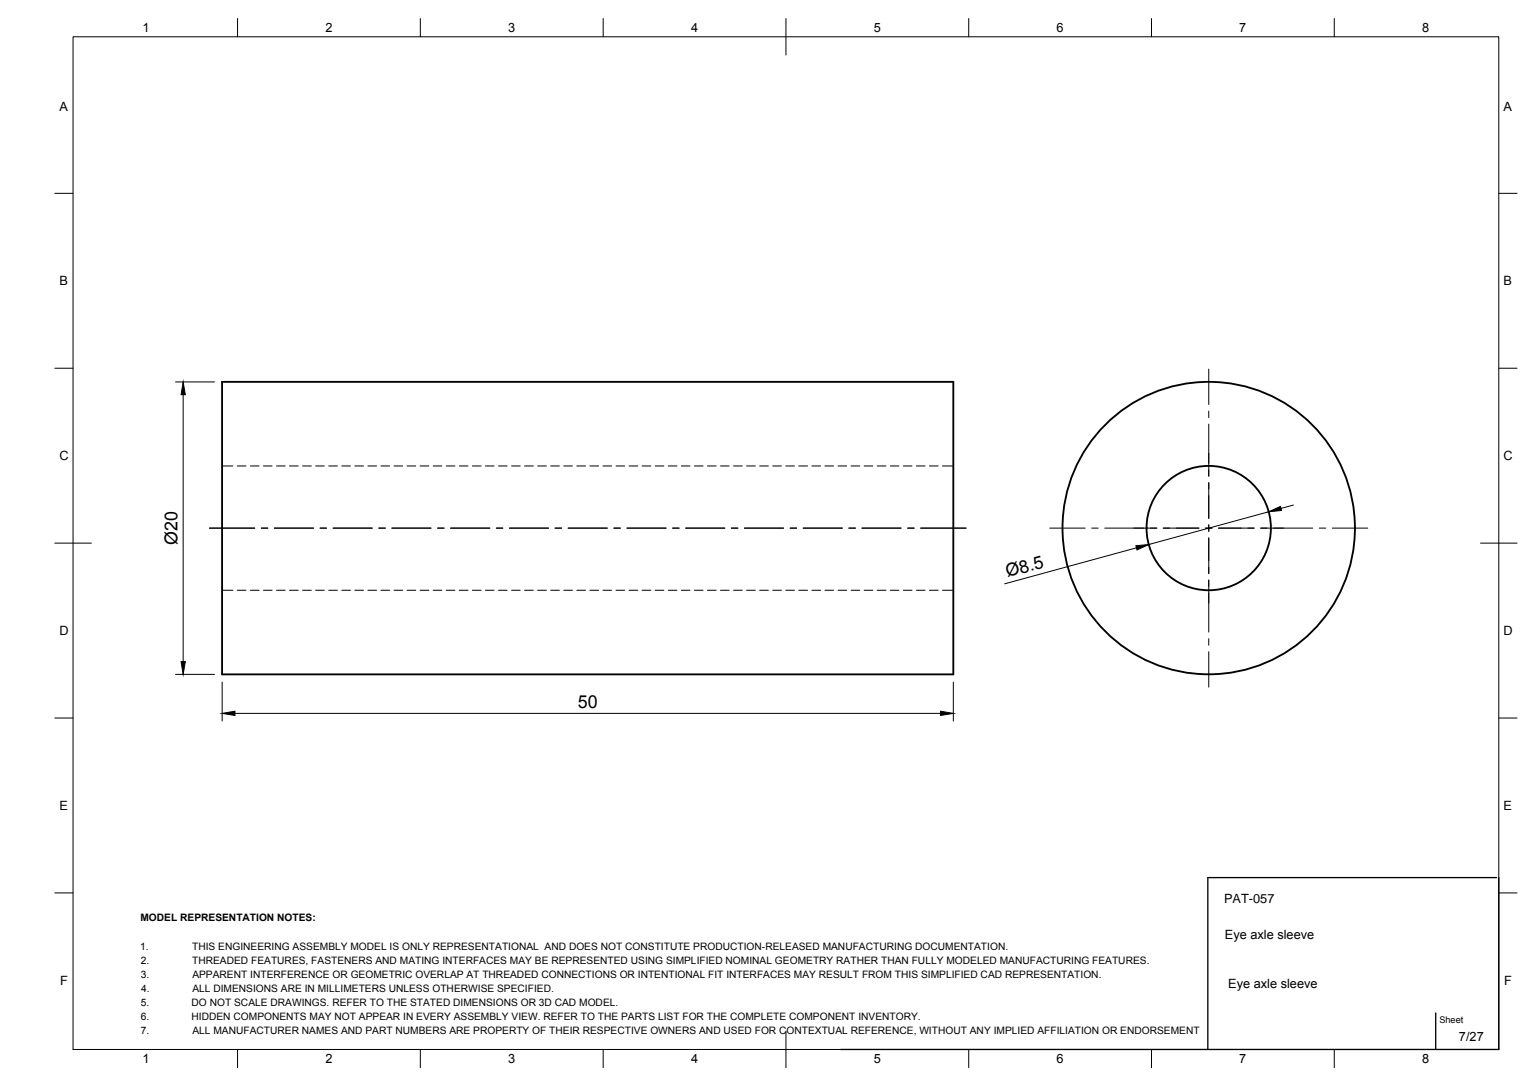
ISO-10303-21;
HEADER;
/* Generated by software containing ST-Developer
 * from STEP Tools, Inc. (www.steptools.com) 
 */

FILE_DESCRIPTION(
/* description */ ('Bearing-mounted hook block'),
/* implementation_level */ '2;1');

FILE_NAME(
/* name */ 'Eye axle sleeve.step',
/* time_stamp */ '2026-10-28T22:30:11-07:00',
/* author */ (''),
/* organization */ (''),
/* preprocessor_version */ 'ST-DEVELOPER v20.2',
/* originating_system */ 'Autodesk Translation Framework v15.17.0.0',
/* authorisation */ '');

FILE_SCHEMA (('AUTOMOTIVE_DESIGN { 1 0 10303 214 3 1 1 }'));
ENDSEC;

DATA;
#10=MECHANICAL_DESIGN_GEOMETRIC_PRESENTATION_REPRESENTATION('',(#325),#7609);
#277=SHAPE_REPRESENTATION_RELATIONSHIP('SRR','None',#7724,#301);
#301=ADVANCED_BREP_SHAPE_REPRESENTATION('',(#357),#7584);
#325=STYLED_ITEM('',(#7931),#357);
#357=MANIFOLD_SOLID_BREP('Body1',#3921);
#440=LINE('',#6266,#670);
#441=LINE('',#6272,#671);
#670=VECTOR('',#4975,0.425);
#671=VECTOR('',#4982,1.);
#860=CYLINDRICAL_SURFACE('',#4298,0.425);
#861=CYLINDRICAL_SURFACE('',#4301,1.);
#941=FACE_BOUND('',#1294,.T.);
#942=FACE_BOUND('',#1296,.T.);
#1035=FACE_OUTER_BOUND('',#1291,.T.);
#1036=FACE_OUTER_BOUND('',#1292,.T.);
#1037=FACE_OUTER_BOUND('',#1293,.T.);
#1038=FACE_OUTER_BOUND('',#1295,.T.);
#1291=EDGE_LOOP('',(#2782,#2783,#2784,#2785));
#1292=EDGE_LOOP('',(#2786,#2787,#2788,#2789));
#1293=EDGE_LOOP('',(#2790));
#1294=EDGE_LOOP('',(#2791));
#1295=EDGE_LOOP('',(#2792));
#1296=EDGE_LOOP('',(#2793));
#1593=CIRCLE('',#4299,0.425);
#1594=CIRCLE('',#4300,0.425);
#1595=CIRCLE('',#4302,1.);
#1596=CIRCLE('',#4303,1.);
#1842=VERTEX_POINT('',#6263);
#1843=VERTEX_POINT('',#6265);
#1844=VERTEX_POINT('',#6269);
#1845=VERTEX_POINT('',#6271);
#2201=EDGE_CURVE('',#1842,#1842,#1593,.T.);
#2202=EDGE_CURVE('',#1842,#1843,#440,.T.);
#2203=EDGE_CURVE('',#1843,#1843,#1594,.T.);
#2204=EDGE_CURVE('',#1844,#1844,#1595,.T.);
#2205=EDGE_CURVE('',#1844,#1845,#441,.T.);
#2206=EDGE_CURVE('',#1845,#1845,#1596,.T.);
#2782=ORIENTED_EDGE('',*,*,#2201,.F.);
#2783=ORIENTED_EDGE('',*,*,#2202,.T.);
#2784=ORIENTED_EDGE('',*,*,#2203,.T.);
#2785=ORIENTED_EDGE('',*,*,#2202,.F.);
#2786=ORIENTED_EDGE('',*,*,#2204,.F.);
#2787=ORIENTED_EDGE('',*,*,#2205,.T.);
#2788=ORIENTED_EDGE('',*,*,#2206,.T.);
#2789=ORIENTED_EDGE('',*,*,#2205,.F.);
#2790=ORIENTED_EDGE('',*,*,#2204,.T.);
#2791=ORIENTED_EDGE('',*,*,#2201,.T.);
#2792=ORIENTED_EDGE('',*,*,#2206,.F.);
#2793=ORIENTED_EDGE('',*,*,#2203,.F.);
#3578=PLANE('',#4304);
#3579=PLANE('',#4305);
#3717=ADVANCED_FACE('',(#1035),#860,.F.);
#3718=ADVANCED_FACE('',(#1036),#861,.T.);
#3719=ADVANCED_FACE('',(#1037,#941),#3578,.T.);
#3720=ADVANCED_FACE('',(#1038,#942),#3579,.F.);
#3921=CLOSED_SHELL('',(#3717,#3718,#3719,#3720));
#4297=AXIS2_PLACEMENT_3D('',#6261,#4969,#4970);
#4298=AXIS2_PLACEMENT_3D('',#6262,#4971,#4972);
#4299=AXIS2_PLACEMENT_3D('',#6264,#4973,#4974);
#4300=AXIS2_PLACEMENT_3D('',#6267,#4976,#4977);
#4301=AXIS2_PLACEMENT_3D('',#6268,#4978,#4979);
#4302=AXIS2_PLACEMENT_3D('',#6270,#4980,#4981);
#4303=AXIS2_PLACEMENT_3D('',#6273,#4983,#4984);
#4304=AXIS2_PLACEMENT_3D('',#6274,#4985,#4986);
#4305=AXIS2_PLACEMENT_3D('',#6275,#4987,#4988);
#4969=DIRECTION('axis',(0.,0.,1.));
#4970=DIRECTION('refdir',(1.,0.,0.));
#4971=DIRECTION('center_axis',(0.,1.,0.));
#4972=DIRECTION('ref_axis',(1.,0.,0.));
#4973=DIRECTION('center_axis',(0.,-1.,0.));
#4974=DIRECTION('ref_axis',(1.,0.,0.));
#4975=DIRECTION('',(0.,-1.,0.));
#4976=DIRECTION('center_axis',(0.,-1.,0.));
#4977=DIRECTION('ref_axis',(1.,0.,0.));
#4978=DIRECTION('center_axis',(0.,1.,0.));
#4979=DIRECTION('ref_axis',(1.,0.,0.));
#4980=DIRECTION('center_axis',(0.,1.,0.));
#4981=DIRECTION('ref_axis',(1.,0.,0.));
#4982=DIRECTION('',(0.,-1.,0.));
#4983=DIRECTION('center_axis',(0.,1.,0.));
#4984=DIRECTION('ref_axis',(1.,0.,0.));
#4985=DIRECTION('center_axis',(0.,1.,0.));
#4986=DIRECTION('ref_axis',(1.,0.,0.));
#4987=DIRECTION('center_axis',(0.,1.,0.));
#4988=DIRECTION('ref_axis',(1.,0.,0.));
#6261=CARTESIAN_POINT('',(0.,0.,0.));
#6262=CARTESIAN_POINT('Origin',(0.,-2.5,20.5));
#6263=CARTESIAN_POINT('',(-0.425,2.5,20.5));
#6264=CARTESIAN_POINT('Origin',(0.,2.5,20.5));
#6265=CARTESIAN_POINT('',(-0.425,-2.5,20.5));
#6266=CARTESIAN_POINT('',(-0.425,-2.5,20.5));
#6267=CARTESIAN_POINT('Origin',(0.,-2.5,20.5));
#6268=CARTESIAN_POINT('Origin',(0.,-2.5,20.5));
#6269=CARTESIAN_POINT('',(-1.,2.5,20.5));
#6270=CARTESIAN_POINT('Origin',(0.,2.5,20.5));
#6271=CARTESIAN_POINT('',(-1.,-2.5,20.5));
#6272=CARTESIAN_POINT('',(-1.,-2.5,20.5));
#6273=CARTESIAN_POINT('Origin',(0.,-2.5,20.5));
#6274=CARTESIAN_POINT('Origin',(0.,2.5,20.5));
#6275=CARTESIAN_POINT('Origin',(0.,-2.5,20.5));
#7554=UNCERTAINTY_MEASURE_WITH_UNIT(LENGTH_MEASURE(0.001),#7610,
'DISTANCE_ACCURACY_VALUE',
'Maximum model space distance between geometric entities at asserted c
onnectivities');
#7579=UNCERTAINTY_MEASURE_WITH_UNIT(LENGTH_MEASURE(0.001),#7610,
'DISTANCE_ACCURACY_VALUE',
'Maximum model space distance between geometric entities at asserted c
onnectivities');
#7584=(
GEOMETRIC_REPRESENTATION_CONTEXT(3)
GLOBAL_UNCERTAINTY_ASSIGNED_CONTEXT((#7554))
GLOBAL_UNIT_ASSIGNED_CONTEXT((#7610,#7612,#7613))
REPRESENTATION_CONTEXT('','3D')
);
#7609=(
GEOMETRIC_REPRESENTATION_CONTEXT(3)
GLOBAL_UNCERTAINTY_ASSIGNED_CONTEXT((#7579))
GLOBAL_UNIT_ASSIGNED_CONTEXT((#7610,#7612,#7613))
REPRESENTATION_CONTEXT('','3D')
);
#7610=(
LENGTH_UNIT()
NAMED_UNIT(*)
SI_UNIT(.CENTI.,.METRE.)
);
#7612=(
NAMED_UNIT(*)
PLANE_ANGLE_UNIT()
SI_UNIT($,.RADIAN.)
);
#7613=(
NAMED_UNIT(*)
SI_UNIT($,.STERADIAN.)
SOLID_ANGLE_UNIT()
);
#7618=SHAPE_DEFINITION_REPRESENTATION(#7647,#7724);
#7647=PRODUCT_DEFINITION_SHAPE('',$,#7754);
#7724=SHAPE_REPRESENTATION('',(#4297),#7584);
#7749=PRODUCT_DEFINITION_CONTEXT('part definition',#7838,'design');
#7754=PRODUCT_DEFINITION('Eye axle sleeve','Eye axle sleeve',#7783,#7749);
#7783=PRODUCT_DEFINITION_FORMATION('',$,#7844);
#7838=APPLICATION_CONTEXT(
'Core Data for Automotive Mechanical Design Process');
#7839=PRODUCT_CONTEXT('part definition',#7838,'mechanical');
#7844=PRODUCT('Eye axle sleeve','Eye axle sleeve','Eye axle sleeve',(#7839));
#7925=COLOUR_RGB('Grey',0.48,0.52,0.57);
#7926=FILL_AREA_STYLE_COLOUR('',#7925);
#7927=FILL_AREA_STYLE('',(#7926));
#7928=SURFACE_STYLE_FILL_AREA(#7927);
#7929=SURFACE_SIDE_STYLE('',(#7928));
#7930=SURFACE_STYLE_USAGE(.BOTH.,#7929);
#7931=PRESENTATION_STYLE_ASSIGNMENT((#7930));
ENDSEC;
END-ISO-10303-21;
